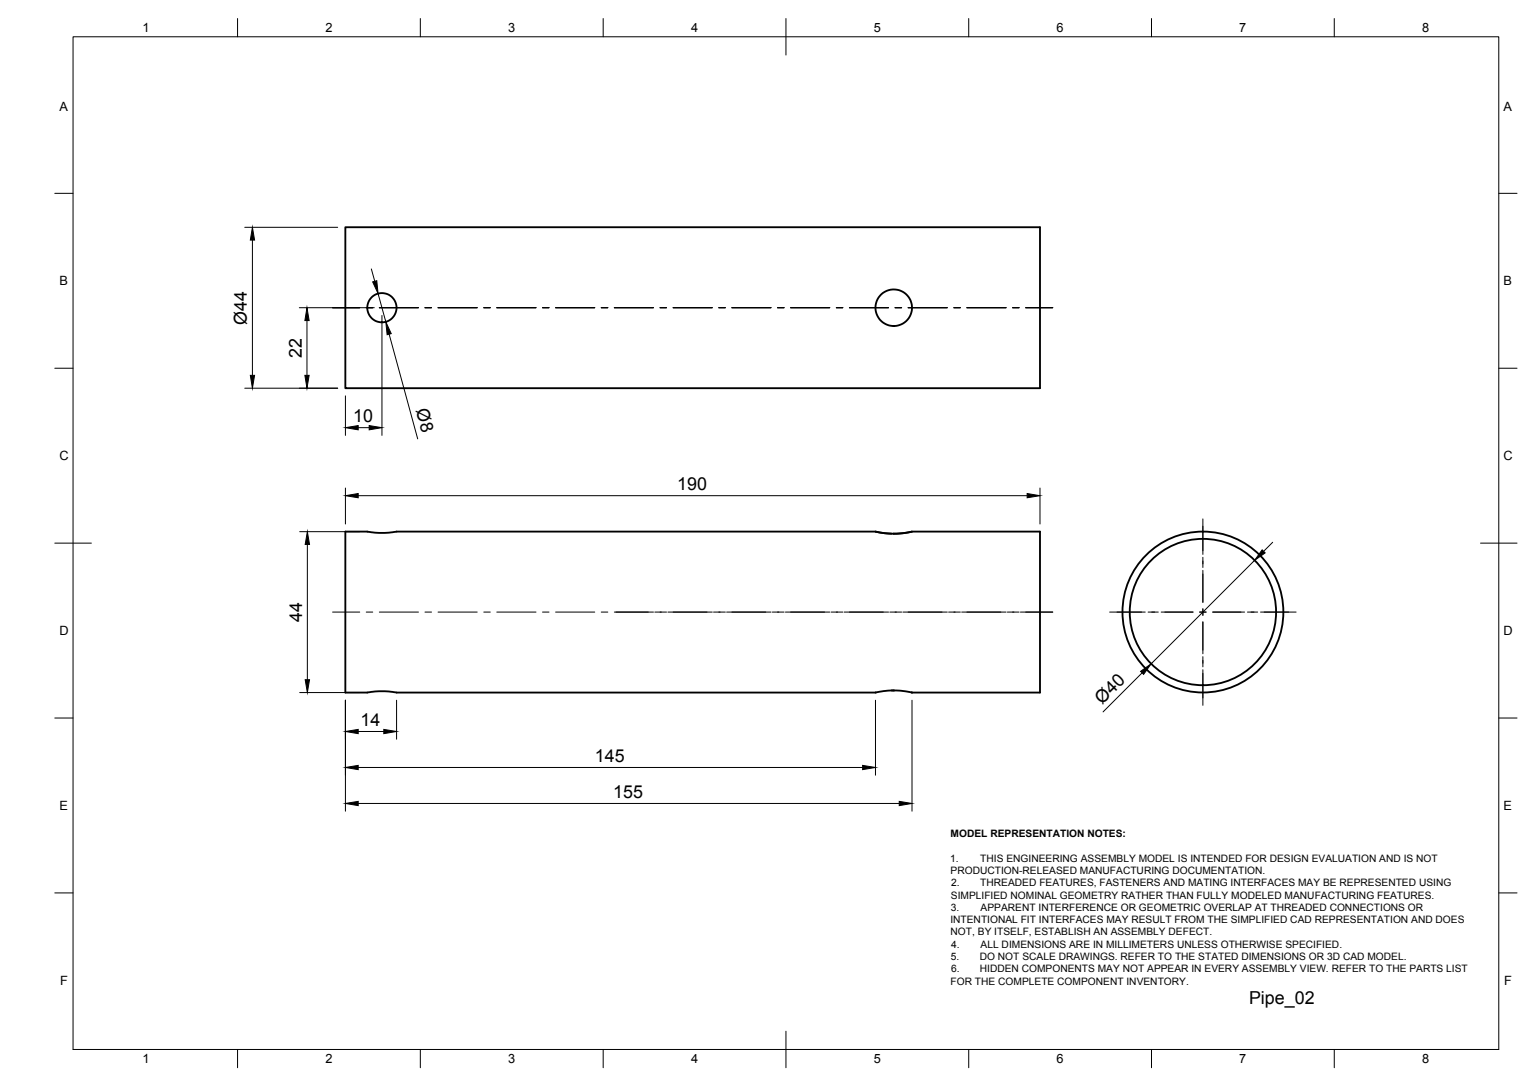
ISO-10303-21;
HEADER;
/* Generated by software containing ST-Developer
 * from STEP Tools, Inc. (www.steptools.com) 
 */

FILE_DESCRIPTION(
/* description */ (''),
/* implementation_level */ '2;1');

FILE_NAME(
/* name */ 'Pipe_02.step',
/* time_stamp */ '2026-10-06T13:31:15-07:00',
/* author */ (''),
/* organization */ (''),
/* preprocessor_version */ 'ST-DEVELOPER v20.2',
/* originating_system */ 'Autodesk Translation Framework v15.15.0.0',
/* authorisation */ '');

FILE_SCHEMA (('AUTOMOTIVE_DESIGN { 1 0 10303 214 3 1 1 }'));
ENDSEC;

DATA;
#10=MECHANICAL_DESIGN_GEOMETRIC_PRESENTATION_REPRESENTATION('',(#87),#3154);
#59=B_SPLINE_SURFACE_WITH_KNOTS('',3,1,((#2777,#2778),(#2779,#2780),(#2781,
#2782),(#2783,#2784),(#2785,#2786),(#2787,#2788),(#2789,#2790),(#2791,#2792),
(#2793,#2794),(#2795,#2796),(#2797,#2798),(#2799,#2800),(#2801,#2802),(#2803,
#2804),(#2805,#2806),(#2807,#2808),(#2809,#2810),(#2811,#2812),(#2813,#2814),
(#2815,#2816),(#2817,#2818),(#2819,#2820),(#2821,#2822),(#2823,#2824),(#2825,
#2826),(#2827,#2828),(#2829,#2830),(#2831,#2832),(#2833,#2834),(#2835,#2836),
(#2837,#2838),(#2839,#2840),(#2841,#2842),(#2843,#2844),(#2845,#2846),(#2847,
#2848),(#2849,#2850)),.UNSPECIFIED.,.T.,.F.,.F.,(4,3,3,3,3,3,3,3,3,3,3,
3,4),(2,2),(-2.41782189489405,-2.24947880033894,-1.98878599548315,-1.8058107663078,
-1.62285095130575,-1.4611068129162,-1.2281083508595,-1.04723806876992,-0.775359720885815,
-0.597430394095587,-0.415845402852008,-0.241029560217643,0.),(0.,28.8022414300165),
 .UNSPECIFIED.);
#60=B_SPLINE_SURFACE_WITH_KNOTS('',3,1,((#2932,#2933),(#2934,#2935),(#2936,
#2937),(#2938,#2939),(#2940,#2941),(#2942,#2943),(#2944,#2945),(#2946,#2947),
(#2948,#2949),(#2950,#2951),(#2952,#2953),(#2954,#2955),(#2956,#2957),(#2958,
#2959),(#2960,#2961),(#2962,#2963),(#2964,#2965),(#2966,#2967),(#2968,#2969),
(#2970,#2971),(#2972,#2973),(#2974,#2975),(#2976,#2977),(#2978,#2979),(#2980,
#2981),(#2982,#2983),(#2984,#2985),(#2986,#2987),(#2988,#2989),(#2990,#2991),
(#2992,#2993),(#2994,#2995),(#2996,#2997),(#2998,#2999),(#3000,#3001),(#3002,
#3003),(#3004,#3005)),.UNSPECIFIED.,.T.,.F.,.F.,(4,3,3,3,3,3,3,3,3,3,3,
3,4),(2,2),(-2.41782189489405,-2.24947880033894,-1.98878599548315,-1.8058107663078,
-1.62285095130575,-1.4611068129162,-1.2281083508595,-1.04723806876992,-0.775359720885815,
-0.597430394095587,-0.415845402852008,-0.241029560217643,0.),(0.,28.8022414300165),
 .UNSPECIFIED.);
#69=SHAPE_REPRESENTATION_RELATIONSHIP('SRR','None',#3197,#78);
#78=ADVANCED_BREP_SHAPE_REPRESENTATION('',(#96),#3153);
#87=STYLED_ITEM('',(#3243),#96);
#96=MANIFOLD_SOLID_BREP('Body1',#1089);
#126=PLANE('',#1269);
#127=PLANE('',#1276);
#133=FACE_BOUND('',#291,.T.);
#134=FACE_BOUND('',#293,.T.);
#135=FACE_BOUND('',#294,.T.);
#136=FACE_BOUND('',#296,.T.);
#137=FACE_BOUND('',#297,.T.);
#138=FACE_BOUND('',#299,.T.);
#167=CIRCLE('',#1270,22.);
#168=CIRCLE('',#1271,20.);
#169=CIRCLE('',#1273,20.);
#170=CIRCLE('',#1275,22.);
#222=FACE_OUTER_BOUND('',#286,.T.);
#223=FACE_OUTER_BOUND('',#287,.T.);
#224=FACE_OUTER_BOUND('',#288,.T.);
#225=FACE_OUTER_BOUND('',#289,.T.);
#226=FACE_OUTER_BOUND('',#290,.T.);
#227=FACE_OUTER_BOUND('',#292,.T.);
#228=FACE_OUTER_BOUND('',#295,.T.);
#229=FACE_OUTER_BOUND('',#298,.T.);
#286=EDGE_LOOP('',(#940,#941,#942,#943,#944,#945));
#287=EDGE_LOOP('',(#946,#947,#948,#949,#950,#951,#952,#953,#954,#955));
#288=EDGE_LOOP('',(#956,#957,#958,#959));
#289=EDGE_LOOP('',(#960,#961,#962,#963,#964,#965,#966,#967));
#290=EDGE_LOOP('',(#968));
#291=EDGE_LOOP('',(#969));
#292=EDGE_LOOP('',(#970,#971,#972,#973,#974,#975,#976,#977,#978,#979,#980,
#981,#982,#983,#984));
#293=EDGE_LOOP('',(#985,#986));
#294=EDGE_LOOP('',(#987));
#295=EDGE_LOOP('',(#988,#989,#990,#991,#992,#993,#994,#995,#996,#997,#998,
#999,#1000,#1001,#1002));
#296=EDGE_LOOP('',(#1003,#1004));
#297=EDGE_LOOP('',(#1005));
#298=EDGE_LOOP('',(#1006));
#299=EDGE_LOOP('',(#1007));
#356=LINE('',#2649,#422);
#357=LINE('',#2723,#423);
#358=LINE('',#2892,#424);
#359=LINE('',#3023,#425);
#360=LINE('',#3112,#426);
#361=LINE('',#3113,#427);
#362=LINE('',#3115,#428);
#363=LINE('',#3120,#429);
#364=LINE('',#3121,#430);
#365=LINE('',#3122,#431);
#422=VECTOR('',#1498,3.99999999999999);
#423=VECTOR('',#1501,3.99999999999999);
#424=VECTOR('',#1502,10.);
#425=VECTOR('',#1503,10.);
#426=VECTOR('',#1512,20.);
#427=VECTOR('',#1513,20.);
#428=VECTOR('',#1514,20.);
#429=VECTOR('',#1521,22.);
#430=VECTOR('',#1522,22.);
#431=VECTOR('',#1523,22.);
#458=B_SPLINE_CURVE_WITH_KNOTS('',3,(#2612,#2613,#2614,#2615,#2616,#2617,
#2618,#2619,#2620,#2621,#2622,#2623,#2624,#2625,#2626,#2627,#2628,#2629),
 .UNSPECIFIED.,.F.,.F.,(4,2,2,2,2,2,2,2,4),(0.,0.15103927001047,0.30207854002094,
0.45311206771438,0.604145595407819,0.755179123101259,0.906212650794699,
1.05725192080517,1.20829119081564),.UNSPECIFIED.);
#459=B_SPLINE_CURVE_WITH_KNOTS('',3,(#2630,#2631,#2632,#2633,#2634,#2635,
#2636,#2637,#2638,#2639,#2640,#2641,#2642,#2643,#2644,#2645,#2646,#2647),
 .UNSPECIFIED.,.F.,.F.,(4,2,2,2,2,2,2,2,4),(1.20829119081564,1.35933046082611,
1.51036973083658,1.66140325853002,1.81243678622346,1.9634703139169,2.11450384161034,
2.26554311162081,2.41658238163128),.UNSPECIFIED.);
#460=B_SPLINE_CURVE_WITH_KNOTS('',3,(#2651,#2652,#2653,#2654,#2655,#2656,
#2657,#2658,#2659,#2660,#2661,#2662,#2663,#2664,#2665,#2666,#2667,#2668),
 .UNSPECIFIED.,.F.,.F.,(4,2,2,2,2,2,2,2,4),(0.,0.151118102356077,0.302236204712155,
0.453345839217834,0.604455473723513,0.755565108229192,0.906674742734871,
1.05779284509095,1.20891094744703),.UNSPECIFIED.);
#461=B_SPLINE_CURVE_WITH_KNOTS('',3,(#2669,#2670,#2671,#2672,#2673,#2674,
#2675,#2676,#2677,#2678,#2679,#2680,#2681,#2682,#2683,#2684,#2685,#2686),
 .UNSPECIFIED.,.F.,.F.,(4,2,2,2,2,2,2,2,4),(1.20891094744703,1.3600290498031,
1.51114715215918,1.66225678666486,1.81336642117054,1.96447605567622,2.1155856901819,
2.26670379253797,2.41782189489405),.UNSPECIFIED.);
#462=B_SPLINE_CURVE_WITH_KNOTS('',3,(#2690,#2691,#2692,#2693,#2694,#2695,
#2696,#2697,#2698,#2699),.UNSPECIFIED.,.F.,.F.,(4,2,2,2,4),(0.,0.151118102356077,
0.302236204712155,0.453345839217834,0.604455473723513),.UNSPECIFIED.);
#463=B_SPLINE_CURVE_WITH_KNOTS('',3,(#2701,#2702,#2703,#2704,#2705,#2706,
#2707,#2708,#2709,#2710),.UNSPECIFIED.,.F.,.F.,(4,2,2,2,4),(1.81336642117054,
1.96447605567622,2.1155856901819,2.26670379253797,2.41782189489405),
 .UNSPECIFIED.);
#464=B_SPLINE_CURVE_WITH_KNOTS('',3,(#2712,#2713,#2714,#2715,#2716,#2717,
#2718,#2719,#2720,#2721),.UNSPECIFIED.,.F.,.F.,(4,2,2,2,4),(1.20891094744703,
1.3600290498031,1.51114715215918,1.66225678666486,1.81336642117054),
 .UNSPECIFIED.);
#465=B_SPLINE_CURVE_WITH_KNOTS('',3,(#2725,#2726,#2727,#2728,#2729,#2730,
#2731,#2732,#2733,#2734),.UNSPECIFIED.,.F.,.F.,(4,2,2,2,4),(0.604145595407819,
0.755179123101259,0.906212650794699,1.05725192080517,1.20829119081564),
 .UNSPECIFIED.);
#466=B_SPLINE_CURVE_WITH_KNOTS('',3,(#2736,#2737,#2738,#2739,#2740,#2741,
#2742,#2743,#2744,#2745),.UNSPECIFIED.,.F.,.F.,(4,2,2,2,4),(0.,0.15103927001047,
0.30207854002094,0.45311206771438,0.604145595407819),.UNSPECIFIED.);
#467=B_SPLINE_CURVE_WITH_KNOTS('',3,(#2747,#2748,#2749,#2750,#2751,#2752,
#2753,#2754,#2755,#2756),.UNSPECIFIED.,.F.,.F.,(4,2,2,2,4),(1.81243678622346,
1.9634703139169,2.11450384161034,2.26554311162081,2.41658238163128),
 .UNSPECIFIED.);
#468=B_SPLINE_CURVE_WITH_KNOTS('',3,(#2757,#2758,#2759,#2760,#2761,#2762,
#2763,#2764,#2765,#2766),.UNSPECIFIED.,.F.,.F.,(4,2,2,2,4),(1.20829119081564,
1.35933046082611,1.51036973083658,1.66140325853002,1.81243678622346),
 .UNSPECIFIED.);
#469=B_SPLINE_CURVE_WITH_KNOTS('',3,(#2767,#2768,#2769,#2770,#2771,#2772,
#2773,#2774,#2775,#2776),.UNSPECIFIED.,.F.,.F.,(4,2,2,2,4),(0.604455473723513,
0.755565108229192,0.906674742734871,1.05779284509095,1.20891094744703),
 .UNSPECIFIED.);
#470=B_SPLINE_CURVE_WITH_KNOTS('',3,(#2852,#2853,#2854,#2855,#2856,#2857,
#2858,#2859,#2860,#2861,#2862,#2863,#2864,#2865,#2866,#2867,#2868,#2869,
#2870,#2871,#2872,#2873,#2874,#2875,#2876,#2877,#2878,#2879,#2880,#2881,
#2882,#2883,#2884,#2885,#2886,#2887,#2888,#2889,#2890),.UNSPECIFIED.,.T.,
 .F.,(4,2,2,2,2,2,2,2,2,3,2,2,2,2,2,2,2,2,4),(-1.22336998493156,-1.09724704826145,
-0.94233260352668,-0.819540701938356,-0.665268805075334,-0.532997978376738,
-0.416879806790855,-0.348119554508441,-0.194082006902748,0.,0.0915534191865666,
0.143556411629729,0.19120578161277,0.250961021394097,0.349888531367616,
0.483105049112713,0.64448257383362,0.847091969730186,0.943107169338909),
 .UNSPECIFIED.);
#471=B_SPLINE_CURVE_WITH_KNOTS('',3,(#2893,#2894,#2895,#2896,#2897,#2898,
#2899,#2900,#2901,#2902,#2903,#2904,#2905,#2906,#2907,#2908,#2909,#2910,
#2911,#2912,#2913,#2914,#2915,#2916,#2917,#2918,#2919,#2920,#2921,#2922,
#2923,#2924,#2925,#2926,#2927,#2928,#2929,#2930,#2931),.UNSPECIFIED.,.T.,
 .F.,(4,2,2,2,2,2,2,2,2,3,2,2,2,2,2,2,2,2,4),(0.841924175679887,0.899224077974559,
1.04154799590402,1.16552064731243,1.2634318988501,1.33413129228483,1.38504379679693,
1.43998123008145,1.50705480177247,1.5985340249232,1.78874148499628,1.89884515666463,
1.94059180293314,2.00808103022965,2.08168057719367,2.18184892200529,2.26512781300167,
2.36548642654063,2.44045820060308),.UNSPECIFIED.);
#472=B_SPLINE_CURVE_WITH_KNOTS('',3,(#3008,#3009,#3010,#3011,#3012,#3013,
#3014,#3015,#3016,#3017,#3018,#3019,#3020,#3021),.UNSPECIFIED.,.F.,.F.,
(4,2,2,2,2,2,4),(-8.38846342825229,-7.81059488838674,-7.33125287845917,
-6.97540830612223,-6.24864745818615,-5.47486898738129,-5.43941055956934),
 .UNSPECIFIED.);
#473=B_SPLINE_CURVE_WITH_KNOTS('',3,(#3025,#3026,#3027,#3028,#3029,#3030,
#3031,#3032,#3033,#3034,#3035,#3036),.UNSPECIFIED.,.F.,.F.,(4,2,2,2,2,4),
(-1.54762978928542,-1.4583177708316,-1.30106672545541,-1.0655082126291,
-0.772398014621137,-0.63986385113685),.UNSPECIFIED.);
#474=B_SPLINE_CURVE_WITH_KNOTS('',3,(#3038,#3039,#3040,#3041,#3042,#3043,
#3044,#3045,#3046,#3047,#3048,#3049,#3050,#3051,#3052,#3053,#3054,#3055,
#3056,#3057,#3058,#3059,#3060),.UNSPECIFIED.,.F.,.F.,(4,2,2,3,2,2,2,2,2,
2,4),(-0.63986385113685,-0.480616814211645,-0.224081253454166,0.,0.120874650966817,
0.237558789133194,0.404814120558448,0.574370503307451,0.750868718798978,
0.951765363187613,1.01851822860381),.UNSPECIFIED.);
#475=B_SPLINE_CURVE_WITH_KNOTS('',3,(#3061,#3062,#3063,#3064,#3065,#3066,
#3067,#3068,#3069,#3070,#3071,#3072),.UNSPECIFIED.,.F.,.F.,(4,2,2,2,2,4),
(1.01851822860381,1.24595614735538,1.70407595255937,2.11785747517733,2.45585059804079,
2.5337692675404),.UNSPECIFIED.);
#476=B_SPLINE_CURVE_WITH_KNOTS('',3,(#3074,#3075,#3076,#3077,#3078,#3079,
#3080,#3081,#3082,#3083,#3084,#3085),.UNSPECIFIED.,.F.,.F.,(4,2,2,2,2,4),
(-1.51818210876971,-1.27085914681692,-1.04616678368018,-0.601418643689676,
-0.233877903034561,-1.0000006369637E-6),.UNSPECIFIED.);
#477=B_SPLINE_CURVE_WITH_KNOTS('',3,(#3086,#3087,#3088,#3089,#3090,#3091,
#3092,#3093,#3094,#3095,#3096,#3097,#3098,#3099,#3100,#3101,#3102,#3103,
#3104,#3105),.UNSPECIFIED.,.F.,.F.,(4,2,2,2,2,2,2,2,2,4),(-5.43941055956934,
-4.53226345790708,-3.19238180995312,-2.23633703092198,-1.64902196252929,
-1.16164668394398,-0.707426447143085,-0.268000268469295,-0.112074736598375,
-9.99999999985594E-7),.UNSPECIFIED.);
#552=VERTEX_POINT('',#2610);
#553=VERTEX_POINT('',#2611);
#554=VERTEX_POINT('',#2648);
#555=VERTEX_POINT('',#2650);
#556=VERTEX_POINT('',#2688);
#557=VERTEX_POINT('',#2689);
#558=VERTEX_POINT('',#2700);
#559=VERTEX_POINT('',#2711);
#560=VERTEX_POINT('',#2722);
#561=VERTEX_POINT('',#2724);
#562=VERTEX_POINT('',#2735);
#563=VERTEX_POINT('',#2746);
#564=VERTEX_POINT('',#2851);
#565=VERTEX_POINT('',#2891);
#566=VERTEX_POINT('',#3006);
#567=VERTEX_POINT('',#3007);
#568=VERTEX_POINT('',#3022);
#569=VERTEX_POINT('',#3024);
#570=VERTEX_POINT('',#3037);
#571=VERTEX_POINT('',#3073);
#572=VERTEX_POINT('',#3107);
#573=VERTEX_POINT('',#3109);
#574=VERTEX_POINT('',#3114);
#575=VERTEX_POINT('',#3118);
#686=EDGE_CURVE('',#552,#553,#458,.T.);
#687=EDGE_CURVE('',#553,#552,#459,.T.);
#688=EDGE_CURVE('',#553,#554,#356,.T.);
#689=EDGE_CURVE('',#555,#554,#460,.T.);
#690=EDGE_CURVE('',#554,#555,#461,.T.);
#691=EDGE_CURVE('',#556,#557,#462,.T.);
#692=EDGE_CURVE('',#558,#556,#463,.T.);
#693=EDGE_CURVE('',#559,#558,#464,.T.);
#694=EDGE_CURVE('',#559,#560,#357,.T.);
#695=EDGE_CURVE('',#561,#560,#465,.T.);
#696=EDGE_CURVE('',#562,#561,#466,.T.);
#697=EDGE_CURVE('',#563,#562,#467,.T.);
#698=EDGE_CURVE('',#560,#563,#468,.T.);
#699=EDGE_CURVE('',#557,#559,#469,.T.);
#700=EDGE_CURVE('',#564,#564,#470,.T.);
#701=EDGE_CURVE('',#564,#565,#358,.T.);
#702=EDGE_CURVE('',#565,#565,#471,.T.);
#703=EDGE_CURVE('',#566,#567,#472,.T.);
#704=EDGE_CURVE('',#568,#566,#359,.T.);
#705=EDGE_CURVE('',#569,#568,#473,.F.);
#706=EDGE_CURVE('',#570,#569,#474,.F.);
#707=EDGE_CURVE('',#568,#570,#475,.F.);
#708=EDGE_CURVE('',#571,#566,#476,.T.);
#709=EDGE_CURVE('',#567,#571,#477,.T.);
#710=EDGE_CURVE('',#572,#572,#167,.T.);
#711=EDGE_CURVE('',#573,#573,#168,.T.);
#712=EDGE_CURVE('',#573,#571,#360,.T.);
#713=EDGE_CURVE('',#567,#558,#361,.T.);
#714=EDGE_CURVE('',#557,#574,#362,.T.);
#715=EDGE_CURVE('',#574,#574,#169,.T.);
#716=EDGE_CURVE('',#575,#575,#170,.T.);
#717=EDGE_CURVE('',#575,#563,#363,.T.);
#718=EDGE_CURVE('',#561,#569,#364,.T.);
#719=EDGE_CURVE('',#570,#572,#365,.T.);
#940=ORIENTED_EDGE('',*,*,#686,.F.);
#941=ORIENTED_EDGE('',*,*,#687,.F.);
#942=ORIENTED_EDGE('',*,*,#688,.T.);
#943=ORIENTED_EDGE('',*,*,#689,.F.);
#944=ORIENTED_EDGE('',*,*,#690,.F.);
#945=ORIENTED_EDGE('',*,*,#688,.F.);
#946=ORIENTED_EDGE('',*,*,#691,.F.);
#947=ORIENTED_EDGE('',*,*,#692,.F.);
#948=ORIENTED_EDGE('',*,*,#693,.F.);
#949=ORIENTED_EDGE('',*,*,#694,.T.);
#950=ORIENTED_EDGE('',*,*,#695,.F.);
#951=ORIENTED_EDGE('',*,*,#696,.F.);
#952=ORIENTED_EDGE('',*,*,#697,.F.);
#953=ORIENTED_EDGE('',*,*,#698,.F.);
#954=ORIENTED_EDGE('',*,*,#694,.F.);
#955=ORIENTED_EDGE('',*,*,#699,.F.);
#956=ORIENTED_EDGE('',*,*,#700,.F.);
#957=ORIENTED_EDGE('',*,*,#701,.T.);
#958=ORIENTED_EDGE('',*,*,#702,.F.);
#959=ORIENTED_EDGE('',*,*,#701,.F.);
#960=ORIENTED_EDGE('',*,*,#703,.F.);
#961=ORIENTED_EDGE('',*,*,#704,.F.);
#962=ORIENTED_EDGE('',*,*,#705,.F.);
#963=ORIENTED_EDGE('',*,*,#706,.F.);
#964=ORIENTED_EDGE('',*,*,#707,.F.);
#965=ORIENTED_EDGE('',*,*,#704,.T.);
#966=ORIENTED_EDGE('',*,*,#708,.F.);
#967=ORIENTED_EDGE('',*,*,#709,.F.);
#968=ORIENTED_EDGE('',*,*,#710,.T.);
#969=ORIENTED_EDGE('',*,*,#711,.T.);
#970=ORIENTED_EDGE('',*,*,#711,.F.);
#971=ORIENTED_EDGE('',*,*,#712,.T.);
#972=ORIENTED_EDGE('',*,*,#708,.T.);
#973=ORIENTED_EDGE('',*,*,#703,.T.);
#974=ORIENTED_EDGE('',*,*,#713,.T.);
#975=ORIENTED_EDGE('',*,*,#692,.T.);
#976=ORIENTED_EDGE('',*,*,#691,.T.);
#977=ORIENTED_EDGE('',*,*,#714,.T.);
#978=ORIENTED_EDGE('',*,*,#715,.F.);
#979=ORIENTED_EDGE('',*,*,#714,.F.);
#980=ORIENTED_EDGE('',*,*,#699,.T.);
#981=ORIENTED_EDGE('',*,*,#693,.T.);
#982=ORIENTED_EDGE('',*,*,#713,.F.);
#983=ORIENTED_EDGE('',*,*,#709,.T.);
#984=ORIENTED_EDGE('',*,*,#712,.F.);
#985=ORIENTED_EDGE('',*,*,#689,.T.);
#986=ORIENTED_EDGE('',*,*,#690,.T.);
#987=ORIENTED_EDGE('',*,*,#700,.T.);
#988=ORIENTED_EDGE('',*,*,#716,.F.);
#989=ORIENTED_EDGE('',*,*,#717,.T.);
#990=ORIENTED_EDGE('',*,*,#697,.T.);
#991=ORIENTED_EDGE('',*,*,#696,.T.);
#992=ORIENTED_EDGE('',*,*,#718,.T.);
#993=ORIENTED_EDGE('',*,*,#705,.T.);
#994=ORIENTED_EDGE('',*,*,#707,.T.);
#995=ORIENTED_EDGE('',*,*,#719,.T.);
#996=ORIENTED_EDGE('',*,*,#710,.F.);
#997=ORIENTED_EDGE('',*,*,#719,.F.);
#998=ORIENTED_EDGE('',*,*,#706,.T.);
#999=ORIENTED_EDGE('',*,*,#718,.F.);
#1000=ORIENTED_EDGE('',*,*,#695,.T.);
#1001=ORIENTED_EDGE('',*,*,#698,.T.);
#1002=ORIENTED_EDGE('',*,*,#717,.F.);
#1003=ORIENTED_EDGE('',*,*,#686,.T.);
#1004=ORIENTED_EDGE('',*,*,#687,.T.);
#1005=ORIENTED_EDGE('',*,*,#702,.T.);
#1006=ORIENTED_EDGE('',*,*,#716,.T.);
#1007=ORIENTED_EDGE('',*,*,#715,.T.);
#1018=CYLINDRICAL_SURFACE('',#1267,3.99999999999999);
#1019=CYLINDRICAL_SURFACE('',#1268,3.99999999999999);
#1020=CYLINDRICAL_SURFACE('',#1272,20.);
#1021=CYLINDRICAL_SURFACE('',#1274,22.);
#1073=ADVANCED_FACE('',(#222),#1018,.F.);
#1074=ADVANCED_FACE('',(#223),#1019,.F.);
#1075=ADVANCED_FACE('',(#224),#59,.F.);
#1076=ADVANCED_FACE('',(#225),#60,.F.);
#1077=ADVANCED_FACE('',(#226,#133),#126,.F.);
#1078=ADVANCED_FACE('',(#227,#134,#135),#1020,.F.);
#1079=ADVANCED_FACE('',(#228,#136,#137),#1021,.T.);
#1080=ADVANCED_FACE('',(#229,#138),#127,.T.);
#1089=CLOSED_SHELL('',(#1073,#1074,#1075,#1076,#1077,#1078,#1079,#1080));
#1266=AXIS2_PLACEMENT_3D('',#2608,#1494,#1495);
#1267=AXIS2_PLACEMENT_3D('',#2609,#1496,#1497);
#1268=AXIS2_PLACEMENT_3D('',#2687,#1499,#1500);
#1269=AXIS2_PLACEMENT_3D('',#3106,#1504,#1505);
#1270=AXIS2_PLACEMENT_3D('',#3108,#1506,#1507);
#1271=AXIS2_PLACEMENT_3D('',#3110,#1508,#1509);
#1272=AXIS2_PLACEMENT_3D('',#3111,#1510,#1511);
#1273=AXIS2_PLACEMENT_3D('',#3116,#1515,#1516);
#1274=AXIS2_PLACEMENT_3D('',#3117,#1517,#1518);
#1275=AXIS2_PLACEMENT_3D('',#3119,#1519,#1520);
#1276=AXIS2_PLACEMENT_3D('',#3123,#1524,#1525);
#1494=DIRECTION('axis',(0.,0.,1.));
#1495=DIRECTION('refdir',(1.,0.,0.));
#1496=DIRECTION('center_axis',(1.,0.,0.));
#1497=DIRECTION('ref_axis',(0.,1.,0.));
#1498=DIRECTION('',(1.,0.,0.));
#1499=DIRECTION('center_axis',(1.,0.,0.));
#1500=DIRECTION('ref_axis',(0.,1.,0.));
#1501=DIRECTION('',(1.,0.,0.));
#1502=DIRECTION('',(-1.,0.,0.));
#1503=DIRECTION('',(-1.,0.,0.));
#1504=DIRECTION('center_axis',(0.,0.,1.));
#1505=DIRECTION('ref_axis',(-1.,0.,0.));
#1506=DIRECTION('center_axis',(0.,0.,-1.));
#1507=DIRECTION('ref_axis',(-1.,0.,0.));
#1508=DIRECTION('center_axis',(0.,0.,1.));
#1509=DIRECTION('ref_axis',(-1.,0.,0.));
#1510=DIRECTION('center_axis',(0.,0.,1.));
#1511=DIRECTION('ref_axis',(-1.,0.,0.));
#1512=DIRECTION('',(0.,0.,1.));
#1513=DIRECTION('',(0.,0.,1.));
#1514=DIRECTION('',(0.,0.,1.));
#1515=DIRECTION('center_axis',(0.,0.,-1.));
#1516=DIRECTION('ref_axis',(-1.,0.,0.));
#1517=DIRECTION('center_axis',(0.,0.,1.));
#1518=DIRECTION('ref_axis',(-1.,0.,0.));
#1519=DIRECTION('center_axis',(0.,0.,1.));
#1520=DIRECTION('ref_axis',(-1.,0.,0.));
#1521=DIRECTION('',(0.,0.,-1.));
#1522=DIRECTION('',(0.,0.,-1.));
#1523=DIRECTION('',(0.,0.,-1.));
#1524=DIRECTION('center_axis',(0.,0.,1.));
#1525=DIRECTION('ref_axis',(-1.,0.,0.));
#2608=CARTESIAN_POINT('',(0.,0.,0.));
#2609=CARTESIAN_POINT('Origin',(-2.,0.,320.));
#2610=CARTESIAN_POINT('',(-21.6333076527839,3.99999999999999,320.));
#2611=CARTESIAN_POINT('',(-21.6333076527839,-3.99999999999999,320.));
#2612=CARTESIAN_POINT('Ctrl Pts',(-21.6333076527839,3.99999999999999,320.));
#2613=CARTESIAN_POINT('Ctrl Pts',(-21.6333076527839,3.99999999999999,320.503464233368));
#2614=CARTESIAN_POINT('Ctrl Pts',(-21.6527030440414,3.8991527689292,321.039701419423));
#2615=CARTESIAN_POINT('Ctrl Pts',(-21.7223085379416,3.49059487648095,322.024875180559));
#2616=CARTESIAN_POINT('Ctrl Pts',(-21.7714644430193,3.18294364927552,322.473910600217));
#2617=CARTESIAN_POINT('Ctrl Pts',(-21.8633822681921,2.47392407847503,323.182930171017));
#2618=CARTESIAN_POINT('Ctrl Pts',(-21.9121811723043,2.02488289993504,323.490591965245));
#2619=CARTESIAN_POINT('Ctrl Pts',(-21.9809663284242,1.03968925279594,323.899157524467));
#2620=CARTESIAN_POINT('Ctrl Pts',(-22.,0.503445092311466,324.));
#2621=CARTESIAN_POINT('Ctrl Pts',(-22.,-0.503445092311465,324.));
#2622=CARTESIAN_POINT('Ctrl Pts',(-21.9809663284242,-1.03968925279593,323.899157524467));
#2623=CARTESIAN_POINT('Ctrl Pts',(-21.9121811723043,-2.02488289993504,323.490591965245));
#2624=CARTESIAN_POINT('Ctrl Pts',(-21.8633822681921,-2.47392407847502,323.182930171017));
#2625=CARTESIAN_POINT('Ctrl Pts',(-21.7714644430193,-3.18294364927552,322.473910600217));
#2626=CARTESIAN_POINT('Ctrl Pts',(-21.7223085379416,-3.49059487648095,322.024875180559));
#2627=CARTESIAN_POINT('Ctrl Pts',(-21.6527030440414,-3.8991527689292,321.039701419423));
#2628=CARTESIAN_POINT('Ctrl Pts',(-21.6333076527839,-3.99999999999999,320.503464233368));
#2629=CARTESIAN_POINT('Ctrl Pts',(-21.6333076527839,-3.99999999999999,320.));
#2630=CARTESIAN_POINT('Ctrl Pts',(-21.6333076527839,-3.99999999999999,320.));
#2631=CARTESIAN_POINT('Ctrl Pts',(-21.6333076527839,-3.99999999999999,319.496535766632));
#2632=CARTESIAN_POINT('Ctrl Pts',(-21.6527030440414,-3.89915276892922,318.960298580577));
#2633=CARTESIAN_POINT('Ctrl Pts',(-21.7223085379416,-3.490594876481,317.975124819441));
#2634=CARTESIAN_POINT('Ctrl Pts',(-21.7714644430193,-3.18294364927552,317.526089399783));
#2635=CARTESIAN_POINT('Ctrl Pts',(-21.8633822681921,-2.47392407847502,316.817069828983));
#2636=CARTESIAN_POINT('Ctrl Pts',(-21.9121811723043,-2.02488289993508,316.509408034755));
#2637=CARTESIAN_POINT('Ctrl Pts',(-21.9809663284242,-1.039689252796,316.100842475533));
#2638=CARTESIAN_POINT('Ctrl Pts',(-22.,-0.503445092311466,316.));
#2639=CARTESIAN_POINT('Ctrl Pts',(-22.,0.503445092311465,316.));
#2640=CARTESIAN_POINT('Ctrl Pts',(-21.9809663284242,1.03968925279597,316.100842475533));
#2641=CARTESIAN_POINT('Ctrl Pts',(-21.9121811723043,2.02488289993506,316.509408034754));
#2642=CARTESIAN_POINT('Ctrl Pts',(-21.8633822681921,2.47392407847503,316.817069828983));
#2643=CARTESIAN_POINT('Ctrl Pts',(-21.7714644430193,3.18294364927552,317.526089399783));
#2644=CARTESIAN_POINT('Ctrl Pts',(-21.7223085379416,3.49059487648096,317.975124819441));
#2645=CARTESIAN_POINT('Ctrl Pts',(-21.6527030440414,3.8991527689292,318.960298580577));
#2646=CARTESIAN_POINT('Ctrl Pts',(-21.6333076527839,3.99999999999999,319.496535766632));
#2647=CARTESIAN_POINT('Ctrl Pts',(-21.6333076527839,3.99999999999999,320.));
#2648=CARTESIAN_POINT('',(-19.5959179422654,-3.99999999999999,320.));
#2649=CARTESIAN_POINT('',(-2.,-3.99999999999999,320.));
#2650=CARTESIAN_POINT('',(-19.5959179422654,3.99999999999999,320.));
#2651=CARTESIAN_POINT('Ctrl Pts',(-19.5959179422654,3.99999999999999,320.));
#2652=CARTESIAN_POINT('Ctrl Pts',(-19.5959179422654,3.99999999999999,319.496272992146));
#2653=CARTESIAN_POINT('Ctrl Pts',(-19.6173550647379,3.89905118499443,318.959928891352));
#2654=CARTESIAN_POINT('Ctrl Pts',(-19.6941660317108,3.4904216705935,317.97483197988));
#2655=CARTESIAN_POINT('Ctrl Pts',(-19.7483634040773,3.18281240876835,317.525958159276));
#2656=CARTESIAN_POINT('Ctrl Pts',(-19.8496135055327,2.47406169858037,316.817207449088));
#2657=CARTESIAN_POINT('Ctrl Pts',(-19.9033338860745,2.02517944479051,316.509582633821));
#2658=CARTESIAN_POINT('Ctrl Pts',(-19.9790475458833,1.04005322432747,316.100941831057));
#2659=CARTESIAN_POINT('Ctrl Pts',(-20.,0.503698781685597,316.));
#2660=CARTESIAN_POINT('Ctrl Pts',(-20.,-0.503698781685597,316.));
#2661=CARTESIAN_POINT('Ctrl Pts',(-19.9790475458833,-1.04005322432746,316.100941831057));
#2662=CARTESIAN_POINT('Ctrl Pts',(-19.9033338860745,-2.02517944479051,316.509582633821));
#2663=CARTESIAN_POINT('Ctrl Pts',(-19.8496135055327,-2.47406169858037,316.817207449088));
#2664=CARTESIAN_POINT('Ctrl Pts',(-19.7483634040773,-3.18281240876835,317.525958159276));
#2665=CARTESIAN_POINT('Ctrl Pts',(-19.6941660317108,-3.49042167059353,317.97483197988));
#2666=CARTESIAN_POINT('Ctrl Pts',(-19.6173550647379,-3.89905118499443,318.959928891352));
#2667=CARTESIAN_POINT('Ctrl Pts',(-19.5959179422654,-3.99999999999999,319.496272992146));
#2668=CARTESIAN_POINT('Ctrl Pts',(-19.5959179422654,-3.99999999999999,320.));
#2669=CARTESIAN_POINT('Ctrl Pts',(-19.5959179422654,-3.99999999999999,320.));
#2670=CARTESIAN_POINT('Ctrl Pts',(-19.5959179422654,-3.99999999999999,320.503727007854));
#2671=CARTESIAN_POINT('Ctrl Pts',(-19.6173550647379,-3.89905118499446,321.040071108647));
#2672=CARTESIAN_POINT('Ctrl Pts',(-19.6941660317108,-3.49042167059358,322.02516802012));
#2673=CARTESIAN_POINT('Ctrl Pts',(-19.7483634040773,-3.18281240876835,322.474041840724));
#2674=CARTESIAN_POINT('Ctrl Pts',(-19.8496135055327,-2.47406169858037,323.182792550912));
#2675=CARTESIAN_POINT('Ctrl Pts',(-19.9033338860745,-2.02517944479054,323.490417366179));
#2676=CARTESIAN_POINT('Ctrl Pts',(-19.9790475458833,-1.04005322432751,323.899058168943));
#2677=CARTESIAN_POINT('Ctrl Pts',(-20.,-0.503698781685598,324.));
#2678=CARTESIAN_POINT('Ctrl Pts',(-20.,0.503698781685596,324.));
#2679=CARTESIAN_POINT('Ctrl Pts',(-19.9790475458833,1.04005322432751,323.899058168943));
#2680=CARTESIAN_POINT('Ctrl Pts',(-19.9033338860745,2.02517944479053,323.490417366179));
#2681=CARTESIAN_POINT('Ctrl Pts',(-19.8496135055327,2.47406169858037,323.182792550912));
#2682=CARTESIAN_POINT('Ctrl Pts',(-19.7483634040773,3.18281240876835,322.474041840724));
#2683=CARTESIAN_POINT('Ctrl Pts',(-19.6941660317108,3.49042167059358,322.02516802012));
#2684=CARTESIAN_POINT('Ctrl Pts',(-19.6173550647379,3.89905118499446,321.040071108647));
#2685=CARTESIAN_POINT('Ctrl Pts',(-19.5959179422654,3.99999999999999,320.503727007854));
#2686=CARTESIAN_POINT('Ctrl Pts',(-19.5959179422654,3.99999999999999,320.));
#2687=CARTESIAN_POINT('Origin',(2.,0.,320.));
#2688=CARTESIAN_POINT('',(19.5959179422654,3.99999999999999,320.));
#2689=CARTESIAN_POINT('',(20.,1.08586892106921E-15,324.));
#2690=CARTESIAN_POINT('Ctrl Pts',(19.5959179422654,3.99999999999999,320.));
#2691=CARTESIAN_POINT('Ctrl Pts',(19.5959179422654,3.99999999999998,320.503727007854));
#2692=CARTESIAN_POINT('Ctrl Pts',(19.6173550647379,3.89905118499446,321.040071108647));
#2693=CARTESIAN_POINT('Ctrl Pts',(19.6941660317108,3.49042167059358,322.02516802012));
#2694=CARTESIAN_POINT('Ctrl Pts',(19.7483634040773,3.18281240876835,322.474041840724));
#2695=CARTESIAN_POINT('Ctrl Pts',(19.8496135055327,2.47406169858037,323.182792550912));
#2696=CARTESIAN_POINT('Ctrl Pts',(19.9033338860745,2.02517944479053,323.490417366179));
#2697=CARTESIAN_POINT('Ctrl Pts',(19.9790475458833,1.04005322432751,323.899058168943));
#2698=CARTESIAN_POINT('Ctrl Pts',(20.,0.503698781685599,324.));
#2699=CARTESIAN_POINT('Ctrl Pts',(20.,2.63677968348475E-15,324.));
#2700=CARTESIAN_POINT('',(20.,4.00020436071024E-15,316.));
#2701=CARTESIAN_POINT('Ctrl Pts',(20.,5.55111512312578E-15,316.));
#2702=CARTESIAN_POINT('Ctrl Pts',(20.,0.503698781685603,316.));
#2703=CARTESIAN_POINT('Ctrl Pts',(19.9790475458833,1.04005322432747,316.100941831057));
#2704=CARTESIAN_POINT('Ctrl Pts',(19.9033338860745,2.02517944479051,316.509582633821));
#2705=CARTESIAN_POINT('Ctrl Pts',(19.8496135055327,2.47406169858037,316.817207449088));
#2706=CARTESIAN_POINT('Ctrl Pts',(19.7483634040773,3.18281240876835,317.525958159276));
#2707=CARTESIAN_POINT('Ctrl Pts',(19.6941660317108,3.4904216705935,317.97483197988));
#2708=CARTESIAN_POINT('Ctrl Pts',(19.6173550647379,3.89905118499443,318.959928891352));
#2709=CARTESIAN_POINT('Ctrl Pts',(19.5959179422654,3.99999999999999,319.496272992146));
#2710=CARTESIAN_POINT('Ctrl Pts',(19.5959179422654,3.99999999999999,320.));
#2711=CARTESIAN_POINT('',(19.5959179422654,-3.99999999999999,320.));
#2712=CARTESIAN_POINT('Ctrl Pts',(19.5959179422654,-3.99999999999999,320.));
#2713=CARTESIAN_POINT('Ctrl Pts',(19.5959179422654,-3.99999999999999,319.496272992146));
#2714=CARTESIAN_POINT('Ctrl Pts',(19.6173550647379,-3.89905118499443,318.959928891352));
#2715=CARTESIAN_POINT('Ctrl Pts',(19.6941660317108,-3.49042167059353,317.97483197988));
#2716=CARTESIAN_POINT('Ctrl Pts',(19.7483634040773,-3.18281240876835,317.525958159276));
#2717=CARTESIAN_POINT('Ctrl Pts',(19.8496135055327,-2.47406169858037,316.817207449088));
#2718=CARTESIAN_POINT('Ctrl Pts',(19.9033338860745,-2.0251794447905,316.509582633821));
#2719=CARTESIAN_POINT('Ctrl Pts',(19.9790475458833,-1.04005322432746,316.100941831057));
#2720=CARTESIAN_POINT('Ctrl Pts',(20.,-0.503698781685596,316.));
#2721=CARTESIAN_POINT('Ctrl Pts',(20.,2.77555756156289E-16,316.));
#2722=CARTESIAN_POINT('',(21.6333076527839,-3.99999999999999,320.));
#2723=CARTESIAN_POINT('',(2.,-3.99999999999999,320.));
#2724=CARTESIAN_POINT('',(22.,2.59611238176539E-15,316.));
#2725=CARTESIAN_POINT('Ctrl Pts',(22.,2.77555756156289E-15,316.));
#2726=CARTESIAN_POINT('Ctrl Pts',(22.,-0.503445092311463,316.));
#2727=CARTESIAN_POINT('Ctrl Pts',(21.9809663284242,-1.03968925279597,316.100842475533));
#2728=CARTESIAN_POINT('Ctrl Pts',(21.9121811723043,-2.02488289993505,316.509408034754));
#2729=CARTESIAN_POINT('Ctrl Pts',(21.8633822681921,-2.47392407847502,316.817069828983));
#2730=CARTESIAN_POINT('Ctrl Pts',(21.7714644430193,-3.18294364927552,317.526089399783));
#2731=CARTESIAN_POINT('Ctrl Pts',(21.7223085379416,-3.49059487648096,317.975124819441));
#2732=CARTESIAN_POINT('Ctrl Pts',(21.6527030440414,-3.8991527689292,318.960298580577));
#2733=CARTESIAN_POINT('Ctrl Pts',(21.6333076527839,-3.99999999999999,319.496535766632));
#2734=CARTESIAN_POINT('Ctrl Pts',(21.6333076527839,-3.99999999999999,320.));
#2735=CARTESIAN_POINT('',(21.6333076527839,4.,320.));
#2736=CARTESIAN_POINT('Ctrl Pts',(21.6333076527839,4.,320.));
#2737=CARTESIAN_POINT('Ctrl Pts',(21.6333076527839,4.,319.496535766632));
#2738=CARTESIAN_POINT('Ctrl Pts',(21.6527030440414,3.8991527689292,318.960298580577));
#2739=CARTESIAN_POINT('Ctrl Pts',(21.7223085379416,3.49059487648096,317.975124819441));
#2740=CARTESIAN_POINT('Ctrl Pts',(21.7714644430193,3.18294364927552,317.526089399783));
#2741=CARTESIAN_POINT('Ctrl Pts',(21.8633822681921,2.47392407847503,316.817069828983));
#2742=CARTESIAN_POINT('Ctrl Pts',(21.9121811723043,2.02488289993506,316.509408034754));
#2743=CARTESIAN_POINT('Ctrl Pts',(21.9809663284242,1.03968925279597,316.100842475533));
#2744=CARTESIAN_POINT('Ctrl Pts',(22.,0.50344509231146,316.));
#2745=CARTESIAN_POINT('Ctrl Pts',(22.,-5.13478148889135E-15,316.));
#2746=CARTESIAN_POINT('',(22.,4.45055271554149E-16,324.));
#2747=CARTESIAN_POINT('Ctrl Pts',(22.,-1.2490009027033E-15,324.));
#2748=CARTESIAN_POINT('Ctrl Pts',(22.,0.503445092311465,324.));
#2749=CARTESIAN_POINT('Ctrl Pts',(21.9809663284242,1.03968925279594,323.899157524467));
#2750=CARTESIAN_POINT('Ctrl Pts',(21.9121811723043,2.02488289993504,323.490591965245));
#2751=CARTESIAN_POINT('Ctrl Pts',(21.8633822681921,2.47392407847503,323.182930171017));
#2752=CARTESIAN_POINT('Ctrl Pts',(21.7714644430193,3.18294364927552,322.473910600217));
#2753=CARTESIAN_POINT('Ctrl Pts',(21.7223085379416,3.49059487648095,322.024875180559));
#2754=CARTESIAN_POINT('Ctrl Pts',(21.6527030440414,3.8991527689292,321.039701419423));
#2755=CARTESIAN_POINT('Ctrl Pts',(21.6333076527839,3.99999999999999,320.503464233368));
#2756=CARTESIAN_POINT('Ctrl Pts',(21.6333076527839,3.99999999999999,320.));
#2757=CARTESIAN_POINT('Ctrl Pts',(21.6333076527839,-3.99999999999999,320.));
#2758=CARTESIAN_POINT('Ctrl Pts',(21.6333076527839,-3.99999999999999,320.503464233368));
#2759=CARTESIAN_POINT('Ctrl Pts',(21.6527030440414,-3.8991527689292,321.039701419423));
#2760=CARTESIAN_POINT('Ctrl Pts',(21.7223085379416,-3.49059487648095,322.024875180559));
#2761=CARTESIAN_POINT('Ctrl Pts',(21.7714644430193,-3.18294364927552,322.473910600217));
#2762=CARTESIAN_POINT('Ctrl Pts',(21.8633822681921,-2.47392407847502,323.182930171017));
#2763=CARTESIAN_POINT('Ctrl Pts',(21.9121811723043,-2.02488289993504,323.490591965245));
#2764=CARTESIAN_POINT('Ctrl Pts',(21.9809663284242,-1.03968925279594,323.899157524467));
#2765=CARTESIAN_POINT('Ctrl Pts',(22.,-0.503445092311467,324.));
#2766=CARTESIAN_POINT('Ctrl Pts',(22.,-1.38777878078145E-15,324.));
#2767=CARTESIAN_POINT('Ctrl Pts',(20.,-2.77555756156289E-16,324.));
#2768=CARTESIAN_POINT('Ctrl Pts',(20.,-0.503698781685597,324.));
#2769=CARTESIAN_POINT('Ctrl Pts',(19.9790475458833,-1.04005322432751,323.899058168943));
#2770=CARTESIAN_POINT('Ctrl Pts',(19.9033338860745,-2.02517944479053,323.490417366179));
#2771=CARTESIAN_POINT('Ctrl Pts',(19.8496135055327,-2.47406169858037,323.182792550912));
#2772=CARTESIAN_POINT('Ctrl Pts',(19.7483634040773,-3.18281240876835,322.474041840724));
#2773=CARTESIAN_POINT('Ctrl Pts',(19.6941660317108,-3.49042167059358,322.02516802012));
#2774=CARTESIAN_POINT('Ctrl Pts',(19.6173550647379,-3.89905118499446,321.040071108647));
#2775=CARTESIAN_POINT('Ctrl Pts',(19.5959179422654,-3.99999999999999,320.503727007854));
#2776=CARTESIAN_POINT('Ctrl Pts',(19.5959179422654,-3.99999999999999,320.));
#2777=CARTESIAN_POINT('Ctrl Pts',(-120.018678583471,4.99999999999999,180.));
#2778=CARTESIAN_POINT('Ctrl Pts',(168.003735716694,4.99999999999999,180.));
#2779=CARTESIAN_POINT('Ctrl Pts',(-120.018678583471,4.99999999999999,180.701429560647));
#2780=CARTESIAN_POINT('Ctrl Pts',(168.003735716694,4.99999999999999,180.701429560647));
#2781=CARTESIAN_POINT('Ctrl Pts',(-120.018678583471,4.84154118145123,181.452551073965));
#2782=CARTESIAN_POINT('Ctrl Pts',(168.003735716694,4.84154118145123,181.452551073965));
#2783=CARTESIAN_POINT('Ctrl Pts',(-120.018678583471,4.52635286465426,182.124177427767));
#2784=CARTESIAN_POINT('Ctrl Pts',(168.003735716694,4.52635286465426,182.124177427767));
#2785=CARTESIAN_POINT('Ctrl Pts',(-120.018678583471,4.03825843713571,183.164244788121));
#2786=CARTESIAN_POINT('Ctrl Pts',(168.003735716694,4.03825843713571,183.164244788121));
#2787=CARTESIAN_POINT('Ctrl Pts',(-120.018678583471,3.23871549390966,183.978582045816));
#2788=CARTESIAN_POINT('Ctrl Pts',(168.003735716694,3.23871549390966,183.978582045816));
#2789=CARTESIAN_POINT('Ctrl Pts',(-120.018678583471,2.20859185585293,184.485768832013));
#2790=CARTESIAN_POINT('Ctrl Pts',(168.003735716694,2.20859185585293,184.485768832013));
#2791=CARTESIAN_POINT('Ctrl Pts',(-120.018678583471,1.4855680314837,184.841753411221));
#2792=CARTESIAN_POINT('Ctrl Pts',(168.003735716694,1.4855680314837,184.841753411221));
#2793=CARTESIAN_POINT('Ctrl Pts',(-120.018678583471,0.672332306955193,185.013639583555));
#2794=CARTESIAN_POINT('Ctrl Pts',(168.003735716694,0.672332306955193,185.013639583555));
#2795=CARTESIAN_POINT('Ctrl Pts',(-120.018678583471,-0.0947408793825885,
184.999102335997));
#2796=CARTESIAN_POINT('Ctrl Pts',(168.003735716694,-0.0947408793825885,
184.999102335997));
#2797=CARTESIAN_POINT('Ctrl Pts',(-120.018678583471,-0.861749446049807,
184.984566313084));
#2798=CARTESIAN_POINT('Ctrl Pts',(168.003735716694,-0.861749446049807,184.984566313084));
#2799=CARTESIAN_POINT('Ctrl Pts',(-120.018678583471,-1.67892656531164,184.777834904611));
#2800=CARTESIAN_POINT('Ctrl Pts',(168.003735716694,-1.67892656531164,184.777834904611));
#2801=CARTESIAN_POINT('Ctrl Pts',(-120.018678583471,-2.38556209111995,184.394211363762));
#2802=CARTESIAN_POINT('Ctrl Pts',(168.003735716694,-2.38556209111995,184.394211363762));
#2803=CARTESIAN_POINT('Ctrl Pts',(-120.018678583471,-3.01025748817222,184.055072088397));
#2804=CARTESIAN_POINT('Ctrl Pts',(168.003735716694,-3.01025748817222,184.055072088397));
#2805=CARTESIAN_POINT('Ctrl Pts',(-120.018678583471,-3.52924546522797,183.609386777));
#2806=CARTESIAN_POINT('Ctrl Pts',(168.003735716694,-3.52924546522797,183.609386777));
#2807=CARTESIAN_POINT('Ctrl Pts',(-120.018678583471,-3.95462292501808,183.059568191906));
#2808=CARTESIAN_POINT('Ctrl Pts',(168.003735716694,-3.95462292501808,183.059568191906));
#2809=CARTESIAN_POINT('Ctrl Pts',(-120.018678583471,-4.56739501624512,182.267534019833));
#2810=CARTESIAN_POINT('Ctrl Pts',(168.003735716694,-4.56739501624512,182.267534019833));
#2811=CARTESIAN_POINT('Ctrl Pts',(-120.018678583471,-4.9464904141789,181.226327567706));
#2812=CARTESIAN_POINT('Ctrl Pts',(168.003735716694,-4.9464904141789,181.226327567706));
#2813=CARTESIAN_POINT('Ctrl Pts',(-120.018678583471,-4.99415183469097,180.241759078532));
#2814=CARTESIAN_POINT('Ctrl Pts',(168.003735716694,-4.99415183469097,180.241759078532));
#2815=CARTESIAN_POINT('Ctrl Pts',(-120.018678583471,-5.03115008136056,179.477465705943));
#2816=CARTESIAN_POINT('Ctrl Pts',(168.003735716694,-5.03115008136056,179.477465705943));
#2817=CARTESIAN_POINT('Ctrl Pts',(-120.018678583471,-4.88912990582069,178.683801029721));
#2818=CARTESIAN_POINT('Ctrl Pts',(168.003735716694,-4.88912990582069,178.683801029721));
#2819=CARTESIAN_POINT('Ctrl Pts',(-120.018678583471,-4.56312148257041,177.956003342639));
#2820=CARTESIAN_POINT('Ctrl Pts',(168.003735716694,-4.56312148257041,177.956003342639));
#2821=CARTESIAN_POINT('Ctrl Pts',(-120.018678583471,-4.07307618333385,176.862001439883));
#2822=CARTESIAN_POINT('Ctrl Pts',(168.003735716694,-4.07307618333385,176.862001439883));
#2823=CARTESIAN_POINT('Ctrl Pts',(-120.018678583471,-3.23595384820037,176.004517412987));
#2824=CARTESIAN_POINT('Ctrl Pts',(168.003735716694,-3.23595384820037,176.004517412987));
#2825=CARTESIAN_POINT('Ctrl Pts',(-120.018678583471,-2.15489635508168,175.488190861876));
#2826=CARTESIAN_POINT('Ctrl Pts',(168.003735716694,-2.15489635508168,175.488190861876));
#2827=CARTESIAN_POINT('Ctrl Pts',(-120.018678583471,-1.44740407601968,175.15028371937));
#2828=CARTESIAN_POINT('Ctrl Pts',(168.003735716694,-1.44740407601968,175.15028371937));
#2829=CARTESIAN_POINT('Ctrl Pts',(-120.018678583471,-0.657548063760293,
174.987640434044));
#2830=CARTESIAN_POINT('Ctrl Pts',(168.003735716694,-0.657548063760293,174.987640434044));
#2831=CARTESIAN_POINT('Ctrl Pts',(-120.018678583471,0.0880693581523543,
175.000775681353));
#2832=CARTESIAN_POINT('Ctrl Pts',(168.003735716694,0.0880693581523543,175.000775681353));
#2833=CARTESIAN_POINT('Ctrl Pts',(-120.018678583471,0.849005936014474,175.014180800174));
#2834=CARTESIAN_POINT('Ctrl Pts',(168.003735716694,0.849005936014474,175.014180800174));
#2835=CARTESIAN_POINT('Ctrl Pts',(-120.018678583471,1.65998081975207,175.216515933084));
#2836=CARTESIAN_POINT('Ctrl Pts',(168.003735716694,1.65998081975207,175.216515933084));
#2837=CARTESIAN_POINT('Ctrl Pts',(-120.018678583471,2.36345091283147,175.593856586238));
#2838=CARTESIAN_POINT('Ctrl Pts',(168.003735716694,2.36345091283147,175.593856586238));
#2839=CARTESIAN_POINT('Ctrl Pts',(-120.018678583471,3.04069695749377,175.957130686094));
#2840=CARTESIAN_POINT('Ctrl Pts',(168.003735716694,3.04069695749377,175.957130686094));
#2841=CARTESIAN_POINT('Ctrl Pts',(-120.018678583471,3.59636505476289,176.445115525822));
#2842=CARTESIAN_POINT('Ctrl Pts',(168.003735716694,3.59636505476289,176.445115525822));
#2843=CARTESIAN_POINT('Ctrl Pts',(-120.018678583471,4.041321668556,177.055900957634));
#2844=CARTESIAN_POINT('Ctrl Pts',(168.003735716694,4.041321668556,177.055900957634));
#2845=CARTESIAN_POINT('Ctrl Pts',(-120.018678583471,4.65481124319825,177.898029118324));
#2846=CARTESIAN_POINT('Ctrl Pts',(168.003735716694,4.65481124319825,177.898029118324));
#2847=CARTESIAN_POINT('Ctrl Pts',(-120.018678583471,4.99999999999999,178.995710165759));
#2848=CARTESIAN_POINT('Ctrl Pts',(168.003735716694,4.99999999999999,178.995710165759));
#2849=CARTESIAN_POINT('Ctrl Pts',(-120.018678583471,4.99999999999999,180.));
#2850=CARTESIAN_POINT('Ctrl Pts',(168.003735716694,4.99999999999999,180.));
#2851=CARTESIAN_POINT('',(-19.3649167310371,4.99999999999999,180.));
#2852=CARTESIAN_POINT('Ctrl Pts',(-19.3649167310371,4.99999999999999,180.));
#2853=CARTESIAN_POINT('Ctrl Pts',(-19.3649167310371,4.99999999999999,179.656276636379));
#2854=CARTESIAN_POINT('Ctrl Pts',(-19.3752683254359,4.96098012900332,179.265182649221));
#2855=CARTESIAN_POINT('Ctrl Pts',(-19.4353496242784,4.72078509063997,178.290368141715));
#2856=CARTESIAN_POINT('Ctrl Pts',(-19.4914325180833,4.50873512303266,177.690061693343));
#2857=CARTESIAN_POINT('Ctrl Pts',(-19.6698374497908,3.64021897653246,176.511459386496));
#2858=CARTESIAN_POINT('Ctrl Pts',(-19.7561738615341,3.167765149487,176.070768115353));
#2859=CARTESIAN_POINT('Ctrl Pts',(-19.9267480044898,1.86096567166663,175.283608655792));
#2860=CARTESIAN_POINT('Ctrl Pts',(-19.9693191762704,1.18642139031165,175.126999474205));
#2861=CARTESIAN_POINT('Ctrl Pts',(-19.9994091583083,0.396121730007714,175.002722388395));
#2862=CARTESIAN_POINT('Ctrl Pts',(-20.0166801524078,-0.277043159907006,
174.932154696418));
#2863=CARTESIAN_POINT('Ctrl Pts',(-19.9244729893901,-1.8944504241017,175.309555396068));
#2864=CARTESIAN_POINT('Ctrl Pts',(-19.8487454717896,-2.4936420409959,175.633241025647));
#2865=CARTESIAN_POINT('Ctrl Pts',(-19.7469625775935,-3.18189012768007,176.126727194768));
#2866=CARTESIAN_POINT('Ctrl Pts',(-19.7059339958017,-3.4246715612765,176.337559801306));
#2867=CARTESIAN_POINT('Ctrl Pts',(-19.5708409016226,-4.15261418047417,177.114358081489));
#2868=CARTESIAN_POINT('Ctrl Pts',(-19.4964574660857,-4.46350630203481,177.693390357527));
#2869=CARTESIAN_POINT('Ctrl Pts',(-19.3986283838268,-4.87322999505193,178.723777174646));
#2870=CARTESIAN_POINT('Ctrl Pts',(-19.3650256499815,-4.99957814958542,179.355073383189));
#2871=CARTESIAN_POINT('Ctrl Pts',(-19.3649475283197,-4.99988072118004,180.002013330726));
#2872=CARTESIAN_POINT('Ctrl Pts',(-19.3649106763447,-5.00002345189721,180.307191359079));
#2873=CARTESIAN_POINT('Ctrl Pts',(-19.3736373833142,-4.97254785920772,180.890223123103));
#2874=CARTESIAN_POINT('Ctrl Pts',(-19.4674269397344,-4.58693311377117,182.017619598821));
#2875=CARTESIAN_POINT('Ctrl Pts',(-19.5183192231322,-4.38551433152747,182.504339680886));
#2876=CARTESIAN_POINT('Ctrl Pts',(-19.6865149822651,-3.55062826109306,183.580157065446));
#2877=CARTESIAN_POINT('Ctrl Pts',(-19.7728418386983,-3.06434838205126,184.009862697332));
#2878=CARTESIAN_POINT('Ctrl Pts',(-19.939001955482,-1.73069169664475,184.767170010893));
#2879=CARTESIAN_POINT('Ctrl Pts',(-19.9761019161117,-1.06408188475894,184.900835849746));
#2880=CARTESIAN_POINT('Ctrl Pts',(-20.0120505317368,0.05230497848514,185.049843619988));
#2881=CARTESIAN_POINT('Ctrl Pts',(-19.9957915020587,0.694184741132029,184.982611117669));
#2882=CARTESIAN_POINT('Ctrl Pts',(-19.9134632202362,2.00564095945725,184.644423471671));
#2883=CARTESIAN_POINT('Ctrl Pts',(-19.8352703571503,2.5969441803465,184.305982645319));
#2884=CARTESIAN_POINT('Ctrl Pts',(-19.6928469146564,3.52972547721907,183.604186924279));
#2885=CARTESIAN_POINT('Ctrl Pts',(-19.6057167803969,3.96687494742429,183.120476018664));
#2886=CARTESIAN_POINT('Ctrl Pts',(-19.4373578240358,4.73060594531999,181.819624478891));
#2887=CARTESIAN_POINT('Ctrl Pts',(-19.3940863845552,4.88606300001282,181.13758993203));
#2888=CARTESIAN_POINT('Ctrl Pts',(-19.3704556074501,4.97859341571146,180.495886648245));
#2889=CARTESIAN_POINT('Ctrl Pts',(-19.3649167310371,4.99999999999999,180.261670622645));
#2890=CARTESIAN_POINT('Ctrl Pts',(-19.3649167310371,4.99999999999999,180.));
#2891=CARTESIAN_POINT('',(-21.4242852856286,4.99999999999999,180.));
#2892=CARTESIAN_POINT('',(-120.018678583471,4.99999999999999,180.));
#2893=CARTESIAN_POINT('Ctrl Pts',(-21.4242852856285,4.99999999999999,180.));
#2894=CARTESIAN_POINT('Ctrl Pts',(-21.4242852856285,4.99999999999999,180.266440972911));
#2895=CARTESIAN_POINT('Ctrl Pts',(-21.4295159134836,4.97766066683645,180.513637485348));
#2896=CARTESIAN_POINT('Ctrl Pts',(-21.4572794964352,4.85725414305748,181.305693804631));
#2897=CARTESIAN_POINT('Ctrl Pts',(-21.5035090198973,4.66401988009852,181.947578824682));
#2898=CARTESIAN_POINT('Ctrl Pts',(-21.6463171087964,3.94382916021953,183.146091812383));
#2899=CARTESIAN_POINT('Ctrl Pts',(-21.7252323873223,3.5068141199092,183.629254356169));
#2900=CARTESIAN_POINT('Ctrl Pts',(-21.8542780588982,2.56268308232979,184.325029328962));
#2901=CARTESIAN_POINT('Ctrl Pts',(-21.9246427130955,1.97682230622835,184.659570461731));
#2902=CARTESIAN_POINT('Ctrl Pts',(-21.9975587820033,0.647370837356641,184.988682812051));
#2903=CARTESIAN_POINT('Ctrl Pts',(-22.0114635671403,0.00763006450754167,
185.052019663629));
#2904=CARTESIAN_POINT('Ctrl Pts',(-21.9724550534794,-1.21362618186779,184.874411158033));
#2905=CARTESIAN_POINT('Ctrl Pts',(-21.932682388788,-1.8531096149277,184.710535799577));
#2906=CARTESIAN_POINT('Ctrl Pts',(-21.7670508838473,-3.27877993846323,183.872852240133));
#2907=CARTESIAN_POINT('Ctrl Pts',(-21.6835800732439,-3.72748016875351,183.362046973031));
#2908=CARTESIAN_POINT('Ctrl Pts',(-21.575660584424,-4.31251978640233,182.58467155384));
#2909=CARTESIAN_POINT('Ctrl Pts',(-21.5217853693328,-4.56550119232117,182.090718612903));
#2910=CARTESIAN_POINT('Ctrl Pts',(-21.4320915723086,-4.9722430980436,180.876072778015));
#2911=CARTESIAN_POINT('Ctrl Pts',(-21.4242940461624,-4.99996246291467,180.30793729798));
#2912=CARTESIAN_POINT('Ctrl Pts',(-21.4243130374363,-4.99988108597961,180.003006565595));
#2913=CARTESIAN_POINT('Ctrl Pts',(-21.4243525248944,-4.99971188362311,179.368981722491));
#2914=CARTESIAN_POINT('Ctrl Pts',(-21.4537490423155,-4.87805507940704,178.732432901037));
#2915=CARTESIAN_POINT('Ctrl Pts',(-21.534494160282,-4.50391537304462,177.797069546953));
#2916=CARTESIAN_POINT('Ctrl Pts',(-21.5996533102872,-4.21889499554481,177.181822069633));
#2917=CARTESIAN_POINT('Ctrl Pts',(-21.7335221221638,-3.42103550068265,176.334952896946));
#2918=CARTESIAN_POINT('Ctrl Pts',(-21.7707205591023,-3.17898668973262,176.123720780895));
#2919=CARTESIAN_POINT('Ctrl Pts',(-21.8626420423699,-2.49167222733435,175.63336844862));
#2920=CARTESIAN_POINT('Ctrl Pts',(-21.9314709722171,-1.89940358158573,175.308986444414));
#2921=CARTESIAN_POINT('Ctrl Pts',(-22.0142761168708,-0.286050077143755,
174.936162313307));
#2922=CARTESIAN_POINT('Ctrl Pts',(-21.9996100525413,0.401172811047044,175.002073703072));
#2923=CARTESIAN_POINT('Ctrl Pts',(-21.9678642907813,1.29586484146865,175.14626218032));
#2924=CARTESIAN_POINT('Ctrl Pts',(-21.9249239566795,1.93920230775896,175.325326856333));
#2925=CARTESIAN_POINT('Ctrl Pts',(-21.7768529503723,3.17624999439771,176.0805697055));
#2926=CARTESIAN_POINT('Ctrl Pts',(-21.6987511052204,3.64994229125153,176.518949199742));
#2927=CARTESIAN_POINT('Ctrl Pts',(-21.5378339057897,4.51120696935556,177.700558030938));
#2928=CARTESIAN_POINT('Ctrl Pts',(-21.4865439748271,4.72726309970277,178.303589812472));
#2929=CARTESIAN_POINT('Ctrl Pts',(-21.433923111627,4.95956788576955,179.269828034558));
#2930=CARTESIAN_POINT('Ctrl Pts',(-21.4242852856285,4.99999999999999,179.651385925244));
#2931=CARTESIAN_POINT('Ctrl Pts',(-21.4242852856285,4.99999999999999,180.));
#2932=CARTESIAN_POINT('Ctrl Pts',(-120.018678583471,4.99999999999999,180.));
#2933=CARTESIAN_POINT('Ctrl Pts',(168.003735716694,4.99999999999999,180.));
#2934=CARTESIAN_POINT('Ctrl Pts',(-120.018678583471,4.99999999999999,180.701429560647));
#2935=CARTESIAN_POINT('Ctrl Pts',(168.003735716694,4.99999999999999,180.701429560647));
#2936=CARTESIAN_POINT('Ctrl Pts',(-120.018678583471,4.84154118145123,181.452551073965));
#2937=CARTESIAN_POINT('Ctrl Pts',(168.003735716694,4.84154118145123,181.452551073965));
#2938=CARTESIAN_POINT('Ctrl Pts',(-120.018678583471,4.52635286465426,182.124177427767));
#2939=CARTESIAN_POINT('Ctrl Pts',(168.003735716694,4.52635286465426,182.124177427767));
#2940=CARTESIAN_POINT('Ctrl Pts',(-120.018678583471,4.03825843713571,183.164244788121));
#2941=CARTESIAN_POINT('Ctrl Pts',(168.003735716694,4.03825843713571,183.164244788121));
#2942=CARTESIAN_POINT('Ctrl Pts',(-120.018678583471,3.23871549390966,183.978582045816));
#2943=CARTESIAN_POINT('Ctrl Pts',(168.003735716694,3.23871549390966,183.978582045816));
#2944=CARTESIAN_POINT('Ctrl Pts',(-120.018678583471,2.20859185585293,184.485768832013));
#2945=CARTESIAN_POINT('Ctrl Pts',(168.003735716694,2.20859185585293,184.485768832013));
#2946=CARTESIAN_POINT('Ctrl Pts',(-120.018678583471,1.4855680314837,184.841753411221));
#2947=CARTESIAN_POINT('Ctrl Pts',(168.003735716694,1.4855680314837,184.841753411221));
#2948=CARTESIAN_POINT('Ctrl Pts',(-120.018678583471,0.672332306955193,185.013639583555));
#2949=CARTESIAN_POINT('Ctrl Pts',(168.003735716694,0.672332306955193,185.013639583555));
#2950=CARTESIAN_POINT('Ctrl Pts',(-120.018678583471,-0.0947408793825885,
184.999102335997));
#2951=CARTESIAN_POINT('Ctrl Pts',(168.003735716694,-0.0947408793825885,
184.999102335997));
#2952=CARTESIAN_POINT('Ctrl Pts',(-120.018678583471,-0.861749446049807,
184.984566313084));
#2953=CARTESIAN_POINT('Ctrl Pts',(168.003735716694,-0.861749446049807,184.984566313084));
#2954=CARTESIAN_POINT('Ctrl Pts',(-120.018678583471,-1.67892656531164,184.777834904611));
#2955=CARTESIAN_POINT('Ctrl Pts',(168.003735716694,-1.67892656531164,184.777834904611));
#2956=CARTESIAN_POINT('Ctrl Pts',(-120.018678583471,-2.38556209111995,184.394211363762));
#2957=CARTESIAN_POINT('Ctrl Pts',(168.003735716694,-2.38556209111995,184.394211363762));
#2958=CARTESIAN_POINT('Ctrl Pts',(-120.018678583471,-3.01025748817222,184.055072088397));
#2959=CARTESIAN_POINT('Ctrl Pts',(168.003735716694,-3.01025748817222,184.055072088397));
#2960=CARTESIAN_POINT('Ctrl Pts',(-120.018678583471,-3.52924546522797,183.609386777));
#2961=CARTESIAN_POINT('Ctrl Pts',(168.003735716694,-3.52924546522797,183.609386777));
#2962=CARTESIAN_POINT('Ctrl Pts',(-120.018678583471,-3.95462292501808,183.059568191906));
#2963=CARTESIAN_POINT('Ctrl Pts',(168.003735716694,-3.95462292501808,183.059568191906));
#2964=CARTESIAN_POINT('Ctrl Pts',(-120.018678583471,-4.56739501624512,182.267534019833));
#2965=CARTESIAN_POINT('Ctrl Pts',(168.003735716694,-4.56739501624512,182.267534019833));
#2966=CARTESIAN_POINT('Ctrl Pts',(-120.018678583471,-4.9464904141789,181.226327567706));
#2967=CARTESIAN_POINT('Ctrl Pts',(168.003735716694,-4.9464904141789,181.226327567706));
#2968=CARTESIAN_POINT('Ctrl Pts',(-120.018678583471,-4.99415183469097,180.241759078532));
#2969=CARTESIAN_POINT('Ctrl Pts',(168.003735716694,-4.99415183469097,180.241759078532));
#2970=CARTESIAN_POINT('Ctrl Pts',(-120.018678583471,-5.03115008136056,179.477465705943));
#2971=CARTESIAN_POINT('Ctrl Pts',(168.003735716694,-5.03115008136056,179.477465705943));
#2972=CARTESIAN_POINT('Ctrl Pts',(-120.018678583471,-4.88912990582069,178.683801029721));
#2973=CARTESIAN_POINT('Ctrl Pts',(168.003735716694,-4.88912990582069,178.683801029721));
#2974=CARTESIAN_POINT('Ctrl Pts',(-120.018678583471,-4.56312148257041,177.956003342639));
#2975=CARTESIAN_POINT('Ctrl Pts',(168.003735716694,-4.56312148257041,177.956003342639));
#2976=CARTESIAN_POINT('Ctrl Pts',(-120.018678583471,-4.07307618333385,176.862001439883));
#2977=CARTESIAN_POINT('Ctrl Pts',(168.003735716694,-4.07307618333385,176.862001439883));
#2978=CARTESIAN_POINT('Ctrl Pts',(-120.018678583471,-3.23595384820037,176.004517412987));
#2979=CARTESIAN_POINT('Ctrl Pts',(168.003735716694,-3.23595384820037,176.004517412987));
#2980=CARTESIAN_POINT('Ctrl Pts',(-120.018678583471,-2.15489635508168,175.488190861876));
#2981=CARTESIAN_POINT('Ctrl Pts',(168.003735716694,-2.15489635508168,175.488190861876));
#2982=CARTESIAN_POINT('Ctrl Pts',(-120.018678583471,-1.44740407601968,175.15028371937));
#2983=CARTESIAN_POINT('Ctrl Pts',(168.003735716694,-1.44740407601968,175.15028371937));
#2984=CARTESIAN_POINT('Ctrl Pts',(-120.018678583471,-0.657548063760293,
174.987640434044));
#2985=CARTESIAN_POINT('Ctrl Pts',(168.003735716694,-0.657548063760293,174.987640434044));
#2986=CARTESIAN_POINT('Ctrl Pts',(-120.018678583471,0.0880693581523543,
175.000775681353));
#2987=CARTESIAN_POINT('Ctrl Pts',(168.003735716694,0.0880693581523543,175.000775681353));
#2988=CARTESIAN_POINT('Ctrl Pts',(-120.018678583471,0.849005936014474,175.014180800174));
#2989=CARTESIAN_POINT('Ctrl Pts',(168.003735716694,0.849005936014474,175.014180800174));
#2990=CARTESIAN_POINT('Ctrl Pts',(-120.018678583471,1.65998081975207,175.216515933084));
#2991=CARTESIAN_POINT('Ctrl Pts',(168.003735716694,1.65998081975207,175.216515933084));
#2992=CARTESIAN_POINT('Ctrl Pts',(-120.018678583471,2.36345091283147,175.593856586238));
#2993=CARTESIAN_POINT('Ctrl Pts',(168.003735716694,2.36345091283147,175.593856586238));
#2994=CARTESIAN_POINT('Ctrl Pts',(-120.018678583471,3.04069695749377,175.957130686094));
#2995=CARTESIAN_POINT('Ctrl Pts',(168.003735716694,3.04069695749377,175.957130686094));
#2996=CARTESIAN_POINT('Ctrl Pts',(-120.018678583471,3.59636505476289,176.445115525822));
#2997=CARTESIAN_POINT('Ctrl Pts',(168.003735716694,3.59636505476289,176.445115525822));
#2998=CARTESIAN_POINT('Ctrl Pts',(-120.018678583471,4.041321668556,177.055900957634));
#2999=CARTESIAN_POINT('Ctrl Pts',(168.003735716694,4.041321668556,177.055900957634));
#3000=CARTESIAN_POINT('Ctrl Pts',(-120.018678583471,4.65481124319825,177.898029118324));
#3001=CARTESIAN_POINT('Ctrl Pts',(168.003735716694,4.65481124319825,177.898029118324));
#3002=CARTESIAN_POINT('Ctrl Pts',(-120.018678583471,4.99999999999999,178.995710165759));
#3003=CARTESIAN_POINT('Ctrl Pts',(168.003735716694,4.99999999999999,178.995710165759));
#3004=CARTESIAN_POINT('Ctrl Pts',(-120.018678583471,4.99999999999999,180.));
#3005=CARTESIAN_POINT('Ctrl Pts',(168.003735716694,4.99999999999999,180.));
#3006=CARTESIAN_POINT('',(19.3649167310371,4.99999999999999,180.));
#3007=CARTESIAN_POINT('',(20.,1.09783585004622E-9,184.999950279416));
#3008=CARTESIAN_POINT('Ctrl Pts',(19.3649167310371,4.99999999999999,180.000000000155));
#3009=CARTESIAN_POINT('Ctrl Pts',(19.3649167310393,4.9999999999915,180.255797976078));
#3010=CARTESIAN_POINT('Ctrl Pts',(19.3709161789166,4.98152900200967,180.815194883544));
#3011=CARTESIAN_POINT('Ctrl Pts',(19.4665112788902,4.5921654017984,182.065094951232));
#3012=CARTESIAN_POINT('Ctrl Pts',(19.5252939307559,4.33900973909425,182.52327366873));
#3013=CARTESIAN_POINT('Ctrl Pts',(19.6155368981629,3.90717831536256,183.14107477953));
#3014=CARTESIAN_POINT('Ctrl Pts',(19.6564128349259,3.69873883889033,183.384935096394));
#3015=CARTESIAN_POINT('Ctrl Pts',(19.7803706292242,2.99455052170116,184.060876404812));
#3016=CARTESIAN_POINT('Ctrl Pts',(19.8559843598647,2.45672095108571,184.394978623011));
#3017=CARTESIAN_POINT('Ctrl Pts',(19.9634978707024,1.33933912050469,184.855602695573));
#3018=CARTESIAN_POINT('Ctrl Pts',(19.9971565484544,0.709366488718439,184.987413058734));
#3019=CARTESIAN_POINT('Ctrl Pts',(19.9999400795374,0.0566981305842219,184.999642855756));
#3020=CARTESIAN_POINT('Ctrl Pts',(19.9999999999969,0.0282649299869405,184.999921943856));
#3021=CARTESIAN_POINT('Ctrl Pts',(20.,2.19566810046035E-9,184.999950279416));
#3022=CARTESIAN_POINT('',(21.4242852856286,4.99999999999999,180.));
#3023=CARTESIAN_POINT('',(-120.018678583471,4.99999999999999,180.));
#3024=CARTESIAN_POINT('',(22.,-1.18558479586405E-15,184.999950279418));
#3025=CARTESIAN_POINT('Ctrl Pts',(21.4242852856286,4.99999999999999,180.));
#3026=CARTESIAN_POINT('Ctrl Pts',(21.4242852856286,5.,180.331321770038));
#3027=CARTESIAN_POINT('Ctrl Pts',(21.4325987305796,4.96571390954325,180.744228596537));
#3028=CARTESIAN_POINT('Ctrl Pts',(21.5061118431463,4.64030421838038,182.04689533232));
#3029=CARTESIAN_POINT('Ctrl Pts',(21.5836207752017,4.26781713536477,182.642067445167));
#3030=CARTESIAN_POINT('Ctrl Pts',(21.7015310022096,3.63232448614424,183.501121906396));
#3031=CARTESIAN_POINT('Ctrl Pts',(21.7809360387086,3.15065181168726,183.942868874243));
#3032=CARTESIAN_POINT('Ctrl Pts',(21.9331646274147,1.85908336411556,184.714255119539));
#3033=CARTESIAN_POINT('Ctrl Pts',(21.9728125131015,1.18137916674032,184.876892121407));
#3034=CARTESIAN_POINT('Ctrl Pts',(21.9944951369469,0.532075416791465,184.974489363689));
#3035=CARTESIAN_POINT('Ctrl Pts',(22.,0.285584181637826,184.999663981717));
#3036=CARTESIAN_POINT('Ctrl Pts',(22.,-1.38777878078145E-15,184.999950279418));
#3037=CARTESIAN_POINT('',(22.,-4.42951769594068E-15,175.000041436246));
#3038=CARTESIAN_POINT('Ctrl Pts',(22.,-3.46944695195361E-17,184.999950279418));
#3039=CARTESIAN_POINT('Ctrl Pts',(22.,-0.343144993886238,185.000294281744));
#3040=CARTESIAN_POINT('Ctrl Pts',(21.9920148363644,-0.742730533301487,184.963404127961));
#3041=CARTESIAN_POINT('Ctrl Pts',(21.9288144272746,-1.90972866300947,184.67667933317));
#3042=CARTESIAN_POINT('Ctrl Pts',(21.861683715817,-2.50617516724031,184.363949860461));
#3043=CARTESIAN_POINT('Ctrl Pts',(21.7448558897055,-3.36520718643722,183.733751683529));
#3044=CARTESIAN_POINT('Ctrl Pts',(21.6678314528203,-3.82957681260466,183.304010209844));
#3045=CARTESIAN_POINT('Ctrl Pts',(21.5909137408081,-4.22284783493632,182.673663309574));
#3046=CARTESIAN_POINT('Ctrl Pts',(21.5494225341618,-4.43498739068646,182.333639499534));
#3047=CARTESIAN_POINT('Ctrl Pts',(21.5124934142766,-4.6075844188304,181.963622213912));
#3048=CARTESIAN_POINT('Ctrl Pts',(21.4569989662757,-4.85934461009825,181.214573663743));
#3049=CARTESIAN_POINT('Ctrl Pts',(21.4365908976517,-4.94710817987512,180.820242962523));
#3050=CARTESIAN_POINT('Ctrl Pts',(21.4166549039084,-5.03285024108842,179.835986416571));
#3051=CARTESIAN_POINT('Ctrl Pts',(21.4300169404193,-4.97942996428264,179.193141115726));
#3052=CARTESIAN_POINT('Ctrl Pts',(21.5179664983127,-4.58460297805858,177.889624577146));
#3053=CARTESIAN_POINT('Ctrl Pts',(21.5872551760404,-4.25995320613274,177.307263465564));
#3054=CARTESIAN_POINT('Ctrl Pts',(21.7294201940974,-3.46441716524137,176.332638954624));
#3055=CARTESIAN_POINT('Ctrl Pts',(21.8081204309277,-2.95990282534955,175.913024012782));
#3056=CARTESIAN_POINT('Ctrl Pts',(21.9452433538611,-1.69304720595882,175.234639236131));
#3057=CARTESIAN_POINT('Ctrl Pts',(21.9816800346771,-1.04378161264859,175.083306187542));
#3058=CARTESIAN_POINT('Ctrl Pts',(21.9981718056279,-0.334310676329425,175.008708067723));
#3059=CARTESIAN_POINT('Ctrl Pts',(22.,-0.163664525260938,175.000188837908));
#3060=CARTESIAN_POINT('Ctrl Pts',(22.,-8.95117313604032E-15,175.000041436246));
#3061=CARTESIAN_POINT('Ctrl Pts',(22.,-8.07513778067204E-15,175.000041436246));
#3062=CARTESIAN_POINT('Ctrl Pts',(22.,0.55763177755329,174.999539214703));
#3063=CARTESIAN_POINT('Ctrl Pts',(21.978779974639,1.03421766230349,175.09619314859));
#3064=CARTESIAN_POINT('Ctrl Pts',(21.907804434142,2.14509079920642,175.419604045985));
#3065=CARTESIAN_POINT('Ctrl Pts',(21.8351237457077,2.71999754273336,175.770662232577));
#3066=CARTESIAN_POINT('Ctrl Pts',(21.7231708721587,3.49905157413913,176.393998413372));
#3067=CARTESIAN_POINT('Ctrl Pts',(21.6453341950524,3.95321208636496,176.838841641996));
#3068=CARTESIAN_POINT('Ctrl Pts',(21.5075642574415,4.63936220273143,178.051649859771));
#3069=CARTESIAN_POINT('Ctrl Pts',(21.4569234677635,4.85895980474394,178.684213723796));
#3070=CARTESIAN_POINT('Ctrl Pts',(21.4305680914706,4.97305062459848,179.483986320334));
#3071=CARTESIAN_POINT('Ctrl Pts',(21.4242852856285,4.99999999999998,179.710944260979));
#3072=CARTESIAN_POINT('Ctrl Pts',(21.4242852856285,4.99999999999999,180.));
#3073=CARTESIAN_POINT('',(20.,3.73185018477662E-8,175.000041436213));
#3074=CARTESIAN_POINT('Ctrl Pts',(20.,3.73185018477662E-8,175.000041436213));
#3075=CARTESIAN_POINT('Ctrl Pts',(19.9999999994719,0.283014742405756,174.999786546055));
#3076=CARTESIAN_POINT('Ctrl Pts',(19.9940509156506,0.605923323897178,175.024997930406));
#3077=CARTESIAN_POINT('Ctrl Pts',(19.9609506136869,1.29116251076544,175.161307989225));
#3078=CARTESIAN_POINT('Ctrl Pts',(19.9372461918188,1.61280644746145,175.258019496083));
#3079=CARTESIAN_POINT('Ctrl Pts',(19.8491448581156,2.5265341012254,175.634358550918));
#3080=CARTESIAN_POINT('Ctrl Pts',(19.7675756297683,3.07602021864376,176.001183353682));
#3081=CARTESIAN_POINT('Ctrl Pts',(19.6164573285741,3.91715832709852,176.845369115547));
#3082=CARTESIAN_POINT('Ctrl Pts',(19.5305943144081,4.31837832508637,177.366881965352));
#3083=CARTESIAN_POINT('Ctrl Pts',(19.4157703435753,4.80263665641219,178.554835809988));
#3084=CARTESIAN_POINT('Ctrl Pts',(19.364916731037,5.,179.220409809718));
#3085=CARTESIAN_POINT('Ctrl Pts',(19.364916731037,4.99999999999999,180.));
#3086=CARTESIAN_POINT('Ctrl Pts',(20.,2.19566825658546E-9,184.999950279416));
#3087=CARTESIAN_POINT('Ctrl Pts',(20.0000000000794,-0.723112919238044,185.000675199334));
#3088=CARTESIAN_POINT('Ctrl Pts',(19.9603313151704,-1.33608862318433,184.8382490823));
#3089=CARTESIAN_POINT('Ctrl Pts',(19.861668819025,-2.43933282825348,184.42152350844));
#3090=CARTESIAN_POINT('Ctrl Pts',(19.7812722460709,-2.98500462201654,184.06136107981));
#3091=CARTESIAN_POINT('Ctrl Pts',(19.6467201921559,-3.75669863207033,183.330111124966));
#3092=CARTESIAN_POINT('Ctrl Pts',(19.5535927557505,-4.21754309036747,182.820222354567));
#3093=CARTESIAN_POINT('Ctrl Pts',(19.420273383868,-4.78563378449318,181.518502203014));
#3094=CARTESIAN_POINT('Ctrl Pts',(19.3701649404359,-4.97966702424725,180.883464015848));
#3095=CARTESIAN_POINT('Ctrl Pts',(19.3613269788473,-5.0139081378988,179.497510292478));
#3096=CARTESIAN_POINT('Ctrl Pts',(19.3893990004176,-4.90922242427567,178.866161431178));
#3097=CARTESIAN_POINT('Ctrl Pts',(19.490023993425,-4.49241017983725,177.727574311806));
#3098=CARTESIAN_POINT('Ctrl Pts',(19.5638224334275,-4.17893232584471,177.169356201936));
#3099=CARTESIAN_POINT('Ctrl Pts',(19.7307171512166,-3.30033088115763,176.183284568005));
#3100=CARTESIAN_POINT('Ctrl Pts',(19.8146316030256,-2.77992493069651,175.792923920205));
#3101=CARTESIAN_POINT('Ctrl Pts',(19.9022548761647,-1.98595529578597,175.405568766714));
#3102=CARTESIAN_POINT('Ctrl Pts',(19.9407500804088,-1.61982691968267,175.242872340369));
#3103=CARTESIAN_POINT('Ctrl Pts',(19.9892865959041,-0.749250106435683,175.044322509877));
#3104=CARTESIAN_POINT('Ctrl Pts',(20.000000000697,-0.373578971202775,175.000377890859));
#3105=CARTESIAN_POINT('Ctrl Pts',(20.,3.73179914053834E-8,175.000041436213));
#3106=CARTESIAN_POINT('Origin',(0.,0.,140.));
#3107=CARTESIAN_POINT('',(22.,2.69422295812418E-15,140.));
#3108=CARTESIAN_POINT('Origin',(0.,0.,140.));
#3109=CARTESIAN_POINT('',(20.,2.44929359829471E-15,140.));
#3110=CARTESIAN_POINT('Origin',(0.,0.,140.));
#3111=CARTESIAN_POINT('Origin',(0.,0.,200.));
#3112=CARTESIAN_POINT('',(20.,2.44929359829471E-15,200.));
#3113=CARTESIAN_POINT('',(20.,2.44929359829471E-15,200.));
#3114=CARTESIAN_POINT('',(20.,2.44929359829471E-15,330.));
#3115=CARTESIAN_POINT('',(20.,2.44929359829471E-15,200.));
#3116=CARTESIAN_POINT('Origin',(0.,0.,330.));
#3117=CARTESIAN_POINT('Origin',(0.,0.,200.));
#3118=CARTESIAN_POINT('',(22.,2.69422295812418E-15,330.));
#3119=CARTESIAN_POINT('Origin',(0.,0.,330.));
#3120=CARTESIAN_POINT('',(22.,2.69422295812418E-15,200.));
#3121=CARTESIAN_POINT('',(22.,2.69422295812418E-15,200.));
#3122=CARTESIAN_POINT('',(22.,2.69422295812418E-15,200.));
#3123=CARTESIAN_POINT('Origin',(0.,0.,330.));
#3142=UNCERTAINTY_MEASURE_WITH_UNIT(LENGTH_MEASURE(0.01),#3155,
'DISTANCE_ACCURACY_VALUE',
'Maximum model space distance between geometric entities at asserted c
onnectivities');
#3143=UNCERTAINTY_MEASURE_WITH_UNIT(LENGTH_MEASURE(0.01),#3155,
'DISTANCE_ACCURACY_VALUE',
'Maximum model space distance between geometric entities at asserted c
onnectivities');
#3153=(
GEOMETRIC_REPRESENTATION_CONTEXT(3)
GLOBAL_UNCERTAINTY_ASSIGNED_CONTEXT((#3142))
GLOBAL_UNIT_ASSIGNED_CONTEXT((#3155,#3157,#3158))
REPRESENTATION_CONTEXT('','3D')
);
#3154=(
GEOMETRIC_REPRESENTATION_CONTEXT(3)
GLOBAL_UNCERTAINTY_ASSIGNED_CONTEXT((#3143))
GLOBAL_UNIT_ASSIGNED_CONTEXT((#3155,#3157,#3158))
REPRESENTATION_CONTEXT('','3D')
);
#3155=(
LENGTH_UNIT()
NAMED_UNIT(*)
SI_UNIT(.MILLI.,.METRE.)
);
#3157=(
NAMED_UNIT(*)
PLANE_ANGLE_UNIT()
SI_UNIT($,.RADIAN.)
);
#3158=(
NAMED_UNIT(*)
SI_UNIT($,.STERADIAN.)
SOLID_ANGLE_UNIT()
);
#3168=SHAPE_DEFINITION_REPRESENTATION(#3178,#3197);
#3178=PRODUCT_DEFINITION_SHAPE('',$,#3208);
#3197=SHAPE_REPRESENTATION('',(#1266),#3153);
#3198=PRODUCT_DEFINITION_CONTEXT('part definition',#3230,'design');
#3208=PRODUCT_DEFINITION('Pipe_02','Pipe_02',#3218,#3198);
#3218=PRODUCT_DEFINITION_FORMATION('',$,#3241);
#3230=APPLICATION_CONTEXT(
'Core Data for Automotive Mechanical Design Process');
#3231=PRODUCT_CONTEXT('part definition',#3230,'mechanical');
#3241=PRODUCT('Pipe_02','Pipe_02',$,(#3231));
#3243=PRESENTATION_STYLE_ASSIGNMENT((#3245));
#3245=SURFACE_STYLE_USAGE(.BOTH.,#3247);
#3247=SURFACE_SIDE_STYLE('',(#3249));
#3249=SURFACE_STYLE_FILL_AREA(#3251);
#3251=FILL_AREA_STYLE('Opaque(160,160,160)',(#3253));
#3253=FILL_AREA_STYLE_COLOUR('Opaque(160,160,160)',#3255);
#3255=COLOUR_RGB('Opaque(160,160,160)', 0.09019608, 0.27058824, 0.51372549);
ENDSEC;
END-ISO-10303-21;
